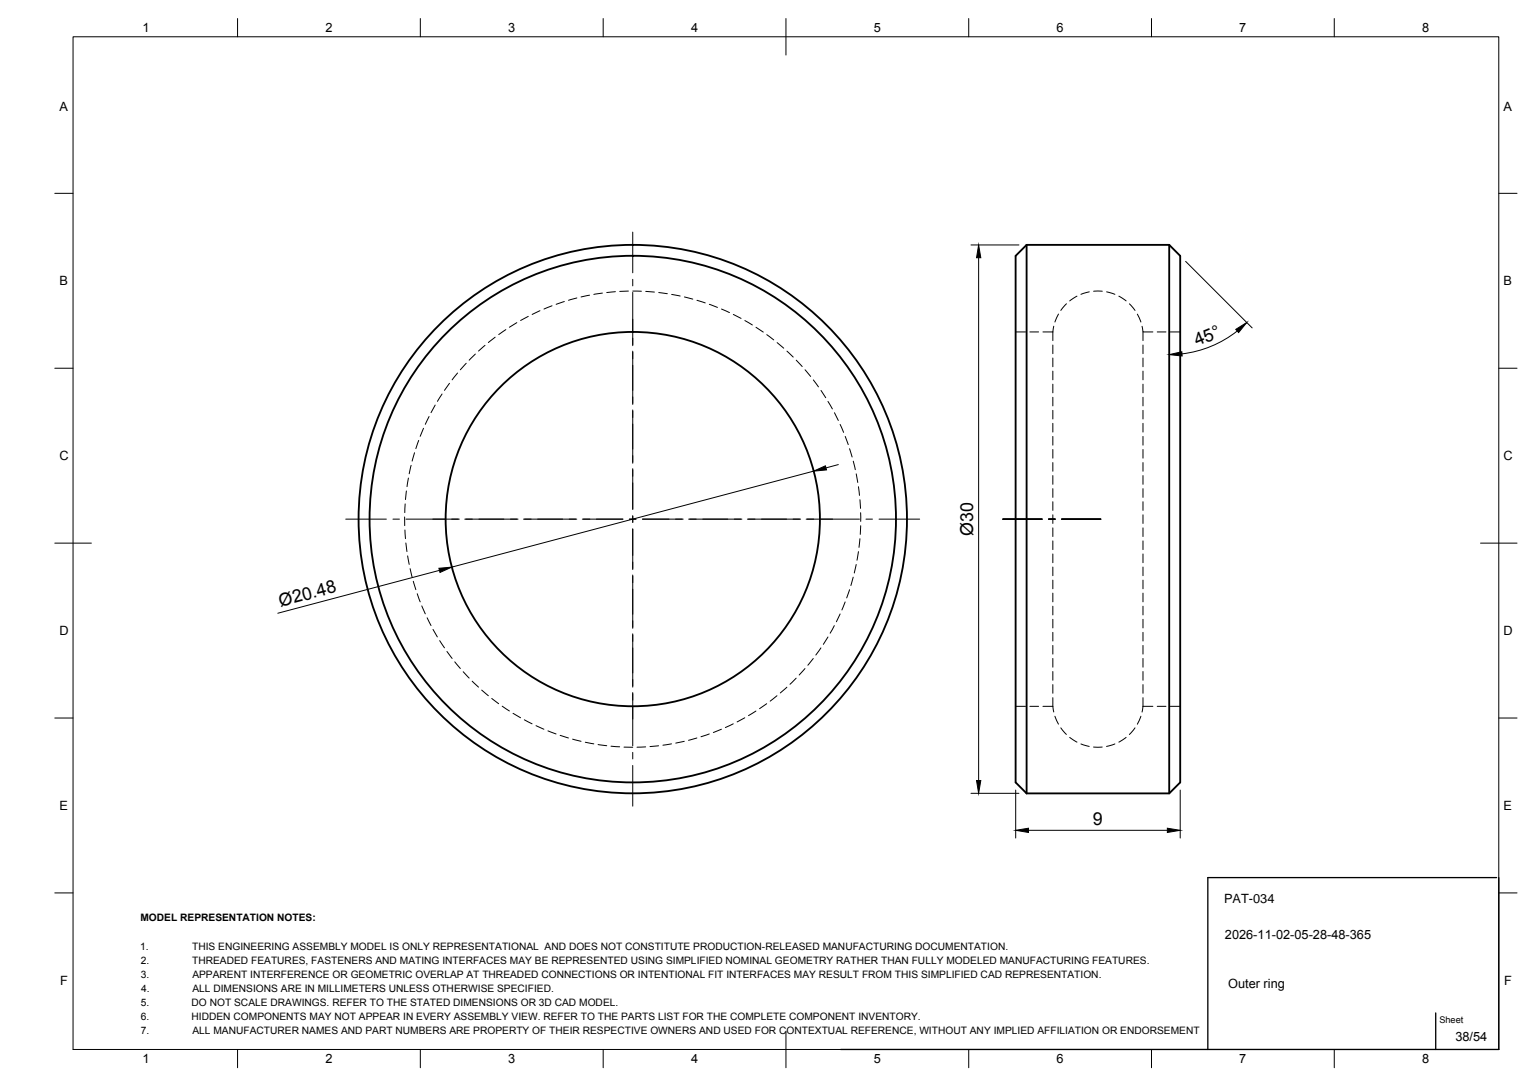
ISO-10303-21;
HEADER;
/* Generated by software containing ST-Developer
 * from STEP Tools, Inc. (www.steptools.com) 
 */

FILE_DESCRIPTION(
/* description */ ('Fatigue rig crank-slider'),
/* implementation_level */ '2;1');

FILE_NAME(
/* name */ 'Outer ring.step',
/* time_stamp */ '2026-10-28T03:24:50-07:00',
/* author */ (''),
/* organization */ (''),
/* preprocessor_version */ 'ST-DEVELOPER v20.2',
/* originating_system */ 'Autodesk Translation Framework v15.17.0.0',
/* authorisation */ '');

FILE_SCHEMA (('AUTOMOTIVE_DESIGN { 1 0 10303 214 3 1 1 }'));
ENDSEC;

DATA;
#10=MECHANICAL_DESIGN_GEOMETRIC_PRESENTATION_REPRESENTATION('',(#621),#16911);
#12=TOROIDAL_SURFACE('',#10128,1.,0.247676);
#24=CONICAL_SURFACE('',#10139,1.47,0.785398163397449);
#25=CONICAL_SURFACE('',#10143,1.47,0.785398163397449);
#520=SHAPE_REPRESENTATION_RELATIONSHIP('SRR','None',#17163,#570);
#570=ADVANCED_BREP_SHAPE_REPRESENTATION('',(#678),#16892);
#621=STYLED_ITEM('',(#17487),#678);
#678=MANIFOLD_SOLID_BREP('Body1',#8914);
#856=FACE_BOUND('',#2232,.T.);
#857=FACE_BOUND('',#2237,.T.);
#1096=PLANE('',#10136);
#1097=PLANE('',#10145);
#1550=FACE_OUTER_BOUND('',#2229,.T.);
#1551=FACE_OUTER_BOUND('',#2230,.T.);
#1552=FACE_OUTER_BOUND('',#2231,.T.);
#1553=FACE_OUTER_BOUND('',#2233,.T.);
#1554=FACE_OUTER_BOUND('',#2234,.T.);
#1555=FACE_OUTER_BOUND('',#2235,.T.);
#1556=FACE_OUTER_BOUND('',#2236,.T.);
#1557=FACE_OUTER_BOUND('',#2238,.T.);
#2229=EDGE_LOOP('',(#7372,#7373,#7374,#7375,#7376,#7377));
#2230=EDGE_LOOP('',(#7378,#7379,#7380,#7381,#7382));
#2231=EDGE_LOOP('',(#7383));
#2232=EDGE_LOOP('',(#7384));
#2233=EDGE_LOOP('',(#7385,#7386,#7387,#7388));
#2234=EDGE_LOOP('',(#7389,#7390,#7391,#7392));
#2235=EDGE_LOOP('',(#7393,#7394,#7395,#7396));
#2236=EDGE_LOOP('',(#7397));
#2237=EDGE_LOOP('',(#7398));
#2238=EDGE_LOOP('',(#7399,#7400,#7401,#7402,#7403));
#2852=LINE('',#15478,#3498);
#2853=LINE('',#15487,#3499);
#2854=LINE('',#15491,#3500);
#2855=LINE('',#15495,#3501);
#2856=LINE('',#15498,#3502);
#3498=VECTOR('',#12244,1.023815);
#3499=VECTOR('',#12255,1.47);
#3500=VECTOR('',#12260,1.5);
#3501=VECTOR('',#12265,1.47);
#3502=VECTOR('',#12270,1.023815);
#4012=CIRCLE('',#10129,1.023815);
#4013=CIRCLE('',#10130,1.023815);
#4014=CIRCLE('',#10131,0.247676);
#4015=CIRCLE('',#10132,1.023815);
#4016=CIRCLE('',#10133,1.023815);
#4017=CIRCLE('',#10135,1.023815);
#4018=CIRCLE('',#10137,1.44);
#4019=CIRCLE('',#10138,1.023815);
#4020=CIRCLE('',#10140,1.5);
#4021=CIRCLE('',#10142,1.5);
#4022=CIRCLE('',#10144,1.44);
#4615=VERTEX_POINT('',#15466);
#4616=VERTEX_POINT('',#15467);
#4617=VERTEX_POINT('',#15470);
#4618=VERTEX_POINT('',#15472);
#4619=VERTEX_POINT('',#15476);
#4620=VERTEX_POINT('',#15480);
#4621=VERTEX_POINT('',#15482);
#4622=VERTEX_POINT('',#15485);
#4623=VERTEX_POINT('',#15489);
#4624=VERTEX_POINT('',#15493);
#5584=EDGE_CURVE('',#4615,#4616,#4012,.T.);
#5585=EDGE_CURVE('',#4616,#4615,#4013,.T.);
#5586=EDGE_CURVE('',#4616,#4617,#4014,.T.);
#5587=EDGE_CURVE('',#4618,#4617,#4015,.T.);
#5588=EDGE_CURVE('',#4617,#4618,#4016,.T.);
#5589=EDGE_CURVE('',#4619,#4619,#4017,.T.);
#5590=EDGE_CURVE('',#4619,#4618,#2852,.T.);
#5591=EDGE_CURVE('',#4620,#4620,#4018,.T.);
#5592=EDGE_CURVE('',#4621,#4621,#4019,.T.);
#5593=EDGE_CURVE('',#4622,#4622,#4020,.T.);
#5594=EDGE_CURVE('',#4622,#4620,#2853,.T.);
#5595=EDGE_CURVE('',#4623,#4623,#4021,.T.);
#5596=EDGE_CURVE('',#4623,#4622,#2854,.T.);
#5597=EDGE_CURVE('',#4624,#4624,#4022,.T.);
#5598=EDGE_CURVE('',#4624,#4623,#2855,.T.);
#5599=EDGE_CURVE('',#4615,#4621,#2856,.T.);
#7372=ORIENTED_EDGE('',*,*,#5584,.F.);
#7373=ORIENTED_EDGE('',*,*,#5585,.F.);
#7374=ORIENTED_EDGE('',*,*,#5586,.T.);
#7375=ORIENTED_EDGE('',*,*,#5587,.F.);
#7376=ORIENTED_EDGE('',*,*,#5588,.F.);
#7377=ORIENTED_EDGE('',*,*,#5586,.F.);
#7378=ORIENTED_EDGE('',*,*,#5589,.T.);
#7379=ORIENTED_EDGE('',*,*,#5590,.T.);
#7380=ORIENTED_EDGE('',*,*,#5587,.T.);
#7381=ORIENTED_EDGE('',*,*,#5588,.T.);
#7382=ORIENTED_EDGE('',*,*,#5590,.F.);
#7383=ORIENTED_EDGE('',*,*,#5591,.F.);
#7384=ORIENTED_EDGE('',*,*,#5592,.T.);
#7385=ORIENTED_EDGE('',*,*,#5593,.F.);
#7386=ORIENTED_EDGE('',*,*,#5594,.T.);
#7387=ORIENTED_EDGE('',*,*,#5591,.T.);
#7388=ORIENTED_EDGE('',*,*,#5594,.F.);
#7389=ORIENTED_EDGE('',*,*,#5595,.F.);
#7390=ORIENTED_EDGE('',*,*,#5596,.T.);
#7391=ORIENTED_EDGE('',*,*,#5593,.T.);
#7392=ORIENTED_EDGE('',*,*,#5596,.F.);
#7393=ORIENTED_EDGE('',*,*,#5597,.F.);
#7394=ORIENTED_EDGE('',*,*,#5598,.T.);
#7395=ORIENTED_EDGE('',*,*,#5595,.T.);
#7396=ORIENTED_EDGE('',*,*,#5598,.F.);
#7397=ORIENTED_EDGE('',*,*,#5597,.T.);
#7398=ORIENTED_EDGE('',*,*,#5589,.F.);
#7399=ORIENTED_EDGE('',*,*,#5584,.T.);
#7400=ORIENTED_EDGE('',*,*,#5585,.T.);
#7401=ORIENTED_EDGE('',*,*,#5599,.T.);
#7402=ORIENTED_EDGE('',*,*,#5592,.F.);
#7403=ORIENTED_EDGE('',*,*,#5599,.F.);
#8316=CYLINDRICAL_SURFACE('',#10134,1.023815);
#8317=CYLINDRICAL_SURFACE('',#10141,1.5);
#8318=CYLINDRICAL_SURFACE('',#10146,1.023815);
#8688=ADVANCED_FACE('',(#1550),#12,.F.);
#8689=ADVANCED_FACE('',(#1551),#8316,.F.);
#8690=ADVANCED_FACE('',(#1552,#856),#1096,.T.);
#8691=ADVANCED_FACE('',(#1553),#24,.T.);
#8692=ADVANCED_FACE('',(#1554),#8317,.T.);
#8693=ADVANCED_FACE('',(#1555),#25,.T.);
#8694=ADVANCED_FACE('',(#1556,#857),#1097,.T.);
#8695=ADVANCED_FACE('',(#1557),#8318,.F.);
#8914=CLOSED_SHELL('',(#8688,#8689,#8690,#8691,#8692,#8693,#8694,#8695));
#10127=AXIS2_PLACEMENT_3D('',#15464,#12226,#12227);
#10128=AXIS2_PLACEMENT_3D('',#15465,#12228,#12229);
#10129=AXIS2_PLACEMENT_3D('',#15468,#12230,#12231);
#10130=AXIS2_PLACEMENT_3D('',#15469,#12232,#12233);
#10131=AXIS2_PLACEMENT_3D('',#15471,#12234,#12235);
#10132=AXIS2_PLACEMENT_3D('',#15473,#12236,#12237);
#10133=AXIS2_PLACEMENT_3D('',#15474,#12238,#12239);
#10134=AXIS2_PLACEMENT_3D('',#15475,#12240,#12241);
#10135=AXIS2_PLACEMENT_3D('',#15477,#12242,#12243);
#10136=AXIS2_PLACEMENT_3D('',#15479,#12245,#12246);
#10137=AXIS2_PLACEMENT_3D('',#15481,#12247,#12248);
#10138=AXIS2_PLACEMENT_3D('',#15483,#12249,#12250);
#10139=AXIS2_PLACEMENT_3D('',#15484,#12251,#12252);
#10140=AXIS2_PLACEMENT_3D('',#15486,#12253,#12254);
#10141=AXIS2_PLACEMENT_3D('',#15488,#12256,#12257);
#10142=AXIS2_PLACEMENT_3D('',#15490,#12258,#12259);
#10143=AXIS2_PLACEMENT_3D('',#15492,#12261,#12262);
#10144=AXIS2_PLACEMENT_3D('',#15494,#12263,#12264);
#10145=AXIS2_PLACEMENT_3D('',#15496,#12266,#12267);
#10146=AXIS2_PLACEMENT_3D('',#15497,#12268,#12269);
#12226=DIRECTION('axis',(0.,0.,1.));
#12227=DIRECTION('refdir',(1.,0.,0.));
#12228=DIRECTION('center_axis',(0.,-1.,0.));
#12229=DIRECTION('ref_axis',(0.,0.,-1.));
#12230=DIRECTION('center_axis',(0.,-1.,0.));
#12231=DIRECTION('ref_axis',(1.,0.,0.));
#12232=DIRECTION('center_axis',(0.,-1.,0.));
#12233=DIRECTION('ref_axis',(1.,0.,0.));
#12234=DIRECTION('center_axis',(1.,0.,1.22464679914735E-16));
#12235=DIRECTION('ref_axis',(-1.22464679914735E-16,0.,1.));
#12236=DIRECTION('center_axis',(0.,1.,0.));
#12237=DIRECTION('ref_axis',(1.,0.,0.));
#12238=DIRECTION('center_axis',(0.,1.,0.));
#12239=DIRECTION('ref_axis',(1.,0.,0.));
#12240=DIRECTION('center_axis',(0.,-1.,0.));
#12241=DIRECTION('ref_axis',(1.,0.,0.));
#12242=DIRECTION('center_axis',(0.,-1.,0.));
#12243=DIRECTION('ref_axis',(1.,0.,0.));
#12244=DIRECTION('',(0.,1.,0.));
#12245=DIRECTION('center_axis',(0.,1.,0.));
#12246=DIRECTION('ref_axis',(0.,0.,1.));
#12247=DIRECTION('center_axis',(0.,-1.,0.));
#12248=DIRECTION('ref_axis',(1.,0.,0.));
#12249=DIRECTION('center_axis',(0.,-1.,0.));
#12250=DIRECTION('ref_axis',(1.,0.,0.));
#12251=DIRECTION('center_axis',(0.,-1.,0.));
#12252=DIRECTION('ref_axis',(1.,0.,0.));
#12253=DIRECTION('center_axis',(0.,-1.,0.));
#12254=DIRECTION('ref_axis',(1.,0.,0.));
#12255=DIRECTION('',(0.707106781186548,0.707106781186547,8.65956056235494E-17));
#12256=DIRECTION('center_axis',(0.,-1.,0.));
#12257=DIRECTION('ref_axis',(1.,0.,0.));
#12258=DIRECTION('center_axis',(0.,-1.,0.));
#12259=DIRECTION('ref_axis',(1.,0.,0.));
#12260=DIRECTION('',(0.,1.,0.));
#12261=DIRECTION('center_axis',(0.,1.,0.));
#12262=DIRECTION('ref_axis',(1.,0.,0.));
#12263=DIRECTION('center_axis',(0.,-1.,0.));
#12264=DIRECTION('ref_axis',(1.,0.,0.));
#12265=DIRECTION('',(-0.707106781186548,0.707106781186547,-8.65956056235494E-17));
#12266=DIRECTION('center_axis',(0.,-1.,0.));
#12267=DIRECTION('ref_axis',(0.,0.,-1.));
#12268=DIRECTION('center_axis',(0.,-1.,0.));
#12269=DIRECTION('ref_axis',(1.,0.,0.));
#12270=DIRECTION('',(0.,1.,0.));
#15464=CARTESIAN_POINT('',(0.,0.,0.));
#15465=CARTESIAN_POINT('Origin',(0.,0.,0.));
#15466=CARTESIAN_POINT('',(-1.023815,0.246528389340863,-1.25381176266905E-16));
#15467=CARTESIAN_POINT('',(-1.25381176266905E-16,0.246528389340863,1.023815));
#15468=CARTESIAN_POINT('Origin',(0.,0.246528389340863,0.));
#15469=CARTESIAN_POINT('Origin',(0.,0.246528389340863,0.));
#15470=CARTESIAN_POINT('',(-1.25381176266905E-16,-0.246528389340863,1.023815));
#15471=CARTESIAN_POINT('Origin',(-1.22464679914735E-16,0.,1.));
#15472=CARTESIAN_POINT('',(-1.023815,-0.246528389340863,1.25381176266905E-16));
#15473=CARTESIAN_POINT('Origin',(0.,-0.246528389340863,0.));
#15474=CARTESIAN_POINT('Origin',(0.,-0.246528389340863,0.));
#15475=CARTESIAN_POINT('Origin',(0.,0.,0.));
#15476=CARTESIAN_POINT('',(-1.023815,-0.45,-1.25381176266905E-16));
#15477=CARTESIAN_POINT('Origin',(0.,-0.45,0.));
#15478=CARTESIAN_POINT('',(-1.023815,0.,-1.25381176266905E-16));
#15479=CARTESIAN_POINT('Origin',(1.44,0.45,0.));
#15480=CARTESIAN_POINT('',(-1.44,0.45,-1.76349139077219E-16));
#15481=CARTESIAN_POINT('Origin',(0.,0.45,0.));
#15482=CARTESIAN_POINT('',(-1.023815,0.45,-1.25381176266905E-16));
#15483=CARTESIAN_POINT('Origin',(0.,0.45,0.));
#15484=CARTESIAN_POINT('Origin',(0.,0.42,0.));
#15485=CARTESIAN_POINT('',(-1.5,0.39,-1.83697019872103E-16));
#15486=CARTESIAN_POINT('Origin',(0.,0.39,0.));
#15487=CARTESIAN_POINT('',(-1.47,0.42,-1.80023079474661E-16));
#15488=CARTESIAN_POINT('Origin',(0.,0.,0.));
#15489=CARTESIAN_POINT('',(-1.5,-0.39,-1.83697019872103E-16));
#15490=CARTESIAN_POINT('Origin',(0.,-0.39,0.));
#15491=CARTESIAN_POINT('',(-1.5,0.,-1.83697019872103E-16));
#15492=CARTESIAN_POINT('Origin',(0.,-0.42,0.));
#15493=CARTESIAN_POINT('',(-1.44,-0.45,-1.76349139077219E-16));
#15494=CARTESIAN_POINT('Origin',(0.,-0.45,0.));
#15495=CARTESIAN_POINT('',(-1.47,-0.42,-1.80023079474661E-16));
#15496=CARTESIAN_POINT('Origin',(1.023815,-0.45,0.));
#15497=CARTESIAN_POINT('Origin',(0.,0.,0.));
#15498=CARTESIAN_POINT('',(-1.023815,0.,-1.25381176266905E-16));
#16833=UNCERTAINTY_MEASURE_WITH_UNIT(LENGTH_MEASURE(0.001),#16912,
'DISTANCE_ACCURACY_VALUE',
'Maximum model space distance between geometric entities at asserted c
onnectivities');
#16852=UNCERTAINTY_MEASURE_WITH_UNIT(LENGTH_MEASURE(0.001),#16912,
'DISTANCE_ACCURACY_VALUE',
'Maximum model space distance between geometric entities at asserted c
onnectivities');
#16892=(
GEOMETRIC_REPRESENTATION_CONTEXT(3)
GLOBAL_UNCERTAINTY_ASSIGNED_CONTEXT((#16833))
GLOBAL_UNIT_ASSIGNED_CONTEXT((#16912,#16914,#16915))
REPRESENTATION_CONTEXT('','3D')
);
#16911=(
GEOMETRIC_REPRESENTATION_CONTEXT(3)
GLOBAL_UNCERTAINTY_ASSIGNED_CONTEXT((#16852))
GLOBAL_UNIT_ASSIGNED_CONTEXT((#16912,#16914,#16915))
REPRESENTATION_CONTEXT('','3D')
);
#16912=(
LENGTH_UNIT()
NAMED_UNIT(*)
SI_UNIT(.CENTI.,.METRE.)
);
#16914=(
NAMED_UNIT(*)
PLANE_ANGLE_UNIT()
SI_UNIT($,.RADIAN.)
);
#16915=(
NAMED_UNIT(*)
SI_UNIT($,.STERADIAN.)
SOLID_ANGLE_UNIT()
);
#16955=SHAPE_DEFINITION_REPRESENTATION(#17015,#17163);
#17015=PRODUCT_DEFINITION_SHAPE('',$,#17222);
#17163=SHAPE_REPRESENTATION('',(#10127),#16892);
#17182=PRODUCT_DEFINITION_CONTEXT('part definition',#17358,'design');
#17222=PRODUCT_DEFINITION('Outer ring','Outer ring',#17280,#17182);
#17280=PRODUCT_DEFINITION_FORMATION('',$,#17399);
#17358=APPLICATION_CONTEXT(
'Core Data for Automotive Mechanical Design Process');
#17359=PRODUCT_CONTEXT('part definition',#17358,'mechanical');
#17399=PRODUCT('Outer ring','Outer ring','Outer ring',(#17359));
#17481=COLOUR_RGB('Grey',0.48,0.52,0.57);
#17482=FILL_AREA_STYLE_COLOUR('',#17481);
#17483=FILL_AREA_STYLE('',(#17482));
#17484=SURFACE_STYLE_FILL_AREA(#17483);
#17485=SURFACE_SIDE_STYLE('',(#17484));
#17486=SURFACE_STYLE_USAGE(.BOTH.,#17485);
#17487=PRESENTATION_STYLE_ASSIGNMENT((#17486));
ENDSEC;
END-ISO-10303-21;
